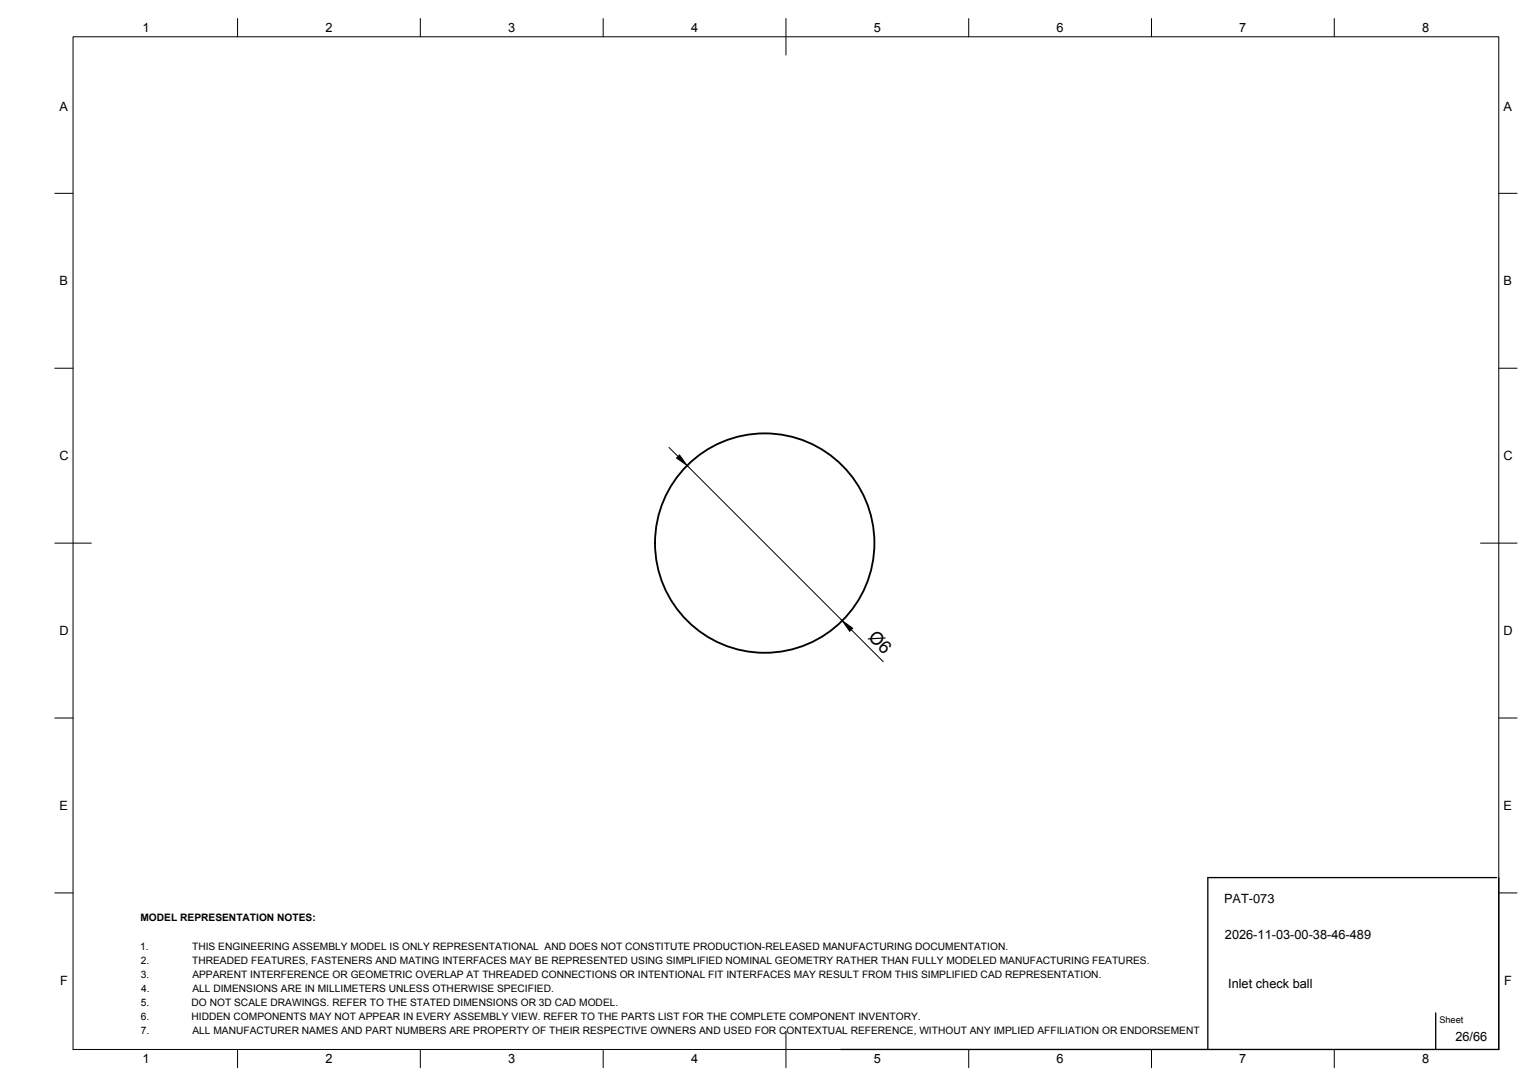
ISO-10303-21;
HEADER;
/* Generated by software containing ST-Developer
 * from STEP Tools, Inc. (www.steptools.com) 
 */

FILE_DESCRIPTION(
/* description */ ('Manual piston pump'),
/* implementation_level */ '2;1');

FILE_NAME(
/* name */ 'Inlet check ball.step',
/* time_stamp */ '2026-11-02T16:54:23-08:00',
/* author */ (''),
/* organization */ (''),
/* preprocessor_version */ 'ST-DEVELOPER v20.2',
/* originating_system */ 'Autodesk Translation Framework v15.17.0.0',
/* authorisation */ '');

FILE_SCHEMA (('AUTOMOTIVE_DESIGN { 1 0 10303 214 3 1 1 }'));
ENDSEC;

DATA;
#10=MECHANICAL_DESIGN_GEOMETRIC_PRESENTATION_REPRESENTATION('',(#726),#19043);
#508=SPHERICAL_SURFACE('',#10952,0.3);
#592=SHAPE_REPRESENTATION_RELATIONSHIP('SRR','None',#19339,#655);
#655=ADVANCED_BREP_SHAPE_REPRESENTATION('',(#796),#19006);
#726=STYLED_ITEM('',(#19661),#796);
#796=MANIFOLD_SOLID_BREP('Body1',#9512);
#1633=FACE_OUTER_BOUND('',#2365,.T.);
#2365=EDGE_LOOP('',(#7699,#7700));
#2985=CIRCLE('',#10953,0.3);
#4834=VERTEX_POINT('',#16643);
#4835=VERTEX_POINT('',#16644);
#5836=EDGE_CURVE('',#4834,#4835,#2985,.T.);
#7699=ORIENTED_EDGE('',*,*,#5836,.T.);
#7700=ORIENTED_EDGE('',*,*,#5836,.F.);
#9238=ADVANCED_FACE('',(#1633),#508,.T.);
#9512=CLOSED_SHELL('',(#9238));
#10951=AXIS2_PLACEMENT_3D('',#16641,#13258,#13259);
#10952=AXIS2_PLACEMENT_3D('',#16642,#13260,#13261);
#10953=AXIS2_PLACEMENT_3D('',#16645,#13262,#13263);
#13258=DIRECTION('axis',(0.,0.,1.));
#13259=DIRECTION('refdir',(1.,0.,0.));
#13260=DIRECTION('center_axis',(0.,0.,1.));
#13261=DIRECTION('ref_axis',(1.,0.,0.));
#13262=DIRECTION('center_axis',(0.,-1.,0.));
#13263=DIRECTION('ref_axis',(-1.,0.,0.));
#16641=CARTESIAN_POINT('',(0.,0.,0.));
#16642=CARTESIAN_POINT('Origin',(-1.5,11.4,8.6));
#16643=CARTESIAN_POINT('',(-1.5,11.4,8.9));
#16644=CARTESIAN_POINT('',(-1.5,11.4,8.3));
#16645=CARTESIAN_POINT('Origin',(-1.5,11.4,8.6));
#18935=UNCERTAINTY_MEASURE_WITH_UNIT(LENGTH_MEASURE(0.001),#19044,
'DISTANCE_ACCURACY_VALUE',
'Maximum model space distance between geometric entities at asserted c
onnectivities');
#18972=UNCERTAINTY_MEASURE_WITH_UNIT(LENGTH_MEASURE(0.001),#19044,
'DISTANCE_ACCURACY_VALUE',
'Maximum model space distance between geometric entities at asserted c
onnectivities');
#19006=(
GEOMETRIC_REPRESENTATION_CONTEXT(3)
GLOBAL_UNCERTAINTY_ASSIGNED_CONTEXT((#18935))
GLOBAL_UNIT_ASSIGNED_CONTEXT((#19044,#19046,#19047))
REPRESENTATION_CONTEXT('','3D')
);
#19043=(
GEOMETRIC_REPRESENTATION_CONTEXT(3)
GLOBAL_UNCERTAINTY_ASSIGNED_CONTEXT((#18972))
GLOBAL_UNIT_ASSIGNED_CONTEXT((#19044,#19046,#19047))
REPRESENTATION_CONTEXT('','3D')
);
#19044=(
LENGTH_UNIT()
NAMED_UNIT(*)
SI_UNIT(.CENTI.,.METRE.)
);
#19046=(
NAMED_UNIT(*)
PLANE_ANGLE_UNIT()
SI_UNIT($,.RADIAN.)
);
#19047=(
NAMED_UNIT(*)
SI_UNIT($,.STERADIAN.)
SOLID_ANGLE_UNIT()
);
#19081=SHAPE_DEFINITION_REPRESENTATION(#19156,#19339);
#19156=PRODUCT_DEFINITION_SHAPE('',$,#19410);
#19339=SHAPE_REPRESENTATION('',(#10951),#19006);
#19376=PRODUCT_DEFINITION_CONTEXT('part definition',#19588,'design');
#19410=PRODUCT_DEFINITION('2026-11-03-00-38-46-489','Inlet check ball',
#19480,#19376);
#19480=PRODUCT_DEFINITION_FORMATION('',$,#19623);
#19588=APPLICATION_CONTEXT(
'Core Data for Automotive Mechanical Design Process');
#19589=PRODUCT_CONTEXT('part definition',#19588,'mechanical');
#19623=PRODUCT('2026-11-03-00-38-46-489','Inlet check ball',
'Inlet check ball',(#19589));
#19661=PRESENTATION_STYLE_ASSIGNMENT((#19667));
#19667=SURFACE_STYLE_USAGE(.BOTH.,#19673);
#19673=SURFACE_SIDE_STYLE('',(#19679));
#19679=SURFACE_STYLE_FILL_AREA(#19685);
#19685=FILL_AREA_STYLE('CAD Library Painted - Engineering blue',(#19691));
#19691=FILL_AREA_STYLE_COLOUR('CAD Library Painted - Engineering blue',
#19697);
#19697=COLOUR_RGB('CAD Library Painted - Engineering blue',0.12156862745098,
0.356862745098039,0.6);
ENDSEC;
END-ISO-10303-21;
